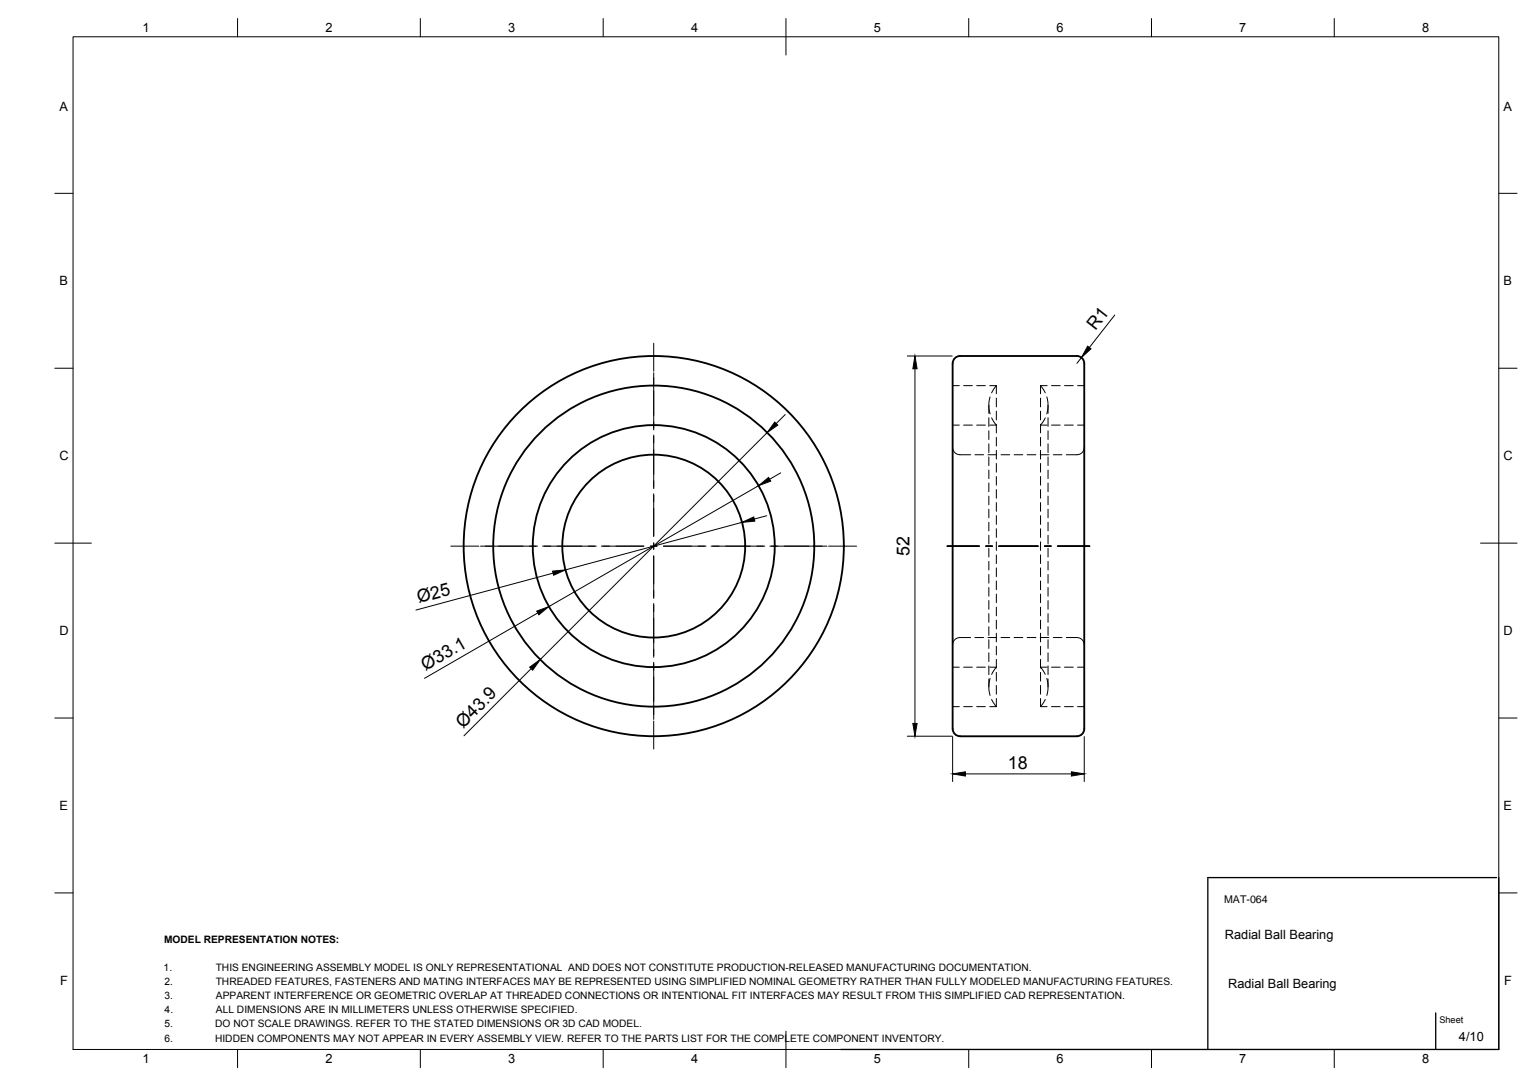
ISO-10303-21;
HEADER;
/* Generated by software containing ST-Developer
 * from STEP Tools, Inc. (www.steptools.com) 
 */

FILE_DESCRIPTION(
/* description */ (''),
/* implementation_level */ '2;1');

FILE_NAME(
/* name */ 
'Radial Ball Bearing.step',
/* time_stamp */ '2026-10-24T12:42:14-07:00',
/* author */ (''),
/* organization */ (''),
/* preprocessor_version */ 'ST-DEVELOPER v20.2',
/* originating_system */ 'Autodesk Translation Framework v15.15.0.0',
/* authorisation */ '');

FILE_SCHEMA (('AUTOMOTIVE_DESIGN { 1 0 10303 214 3 1 1 }'));
ENDSEC;

DATA;
#10=MECHANICAL_DESIGN_GEOMETRIC_PRESENTATION_REPRESENTATION('',(#69),#6789);
#57=SHAPE_REPRESENTATION_RELATIONSHIP('SRR','None',#6824,#63);
#63=ADVANCED_BREP_SHAPE_REPRESENTATION('',(#75),#6786);
#69=STYLED_ITEM('',(#6863),#75);
#75=MANIFOLD_SOLID_BREP('Radial Ball Bearing',#3964);
#86=TOROIDAL_SURFACE('',#4310,19.25,4.05);
#87=TOROIDAL_SURFACE('',#4324,13.5,1.);
#88=TOROIDAL_SURFACE('',#4329,13.5,1.);
#89=TOROIDAL_SURFACE('',#4333,19.25,4.05);
#90=TOROIDAL_SURFACE('',#4343,25.,0.999999999999999);
#91=TOROIDAL_SURFACE('',#4348,25.,0.999999999999999);
#161=CYLINDRICAL_SURFACE('',#4316,16.55);
#162=CYLINDRICAL_SURFACE('',#4318,16.55);
#163=CYLINDRICAL_SURFACE('',#4327,12.5);
#164=CYLINDRICAL_SURFACE('',#4337,21.95);
#165=CYLINDRICAL_SURFACE('',#4339,21.95);
#166=CYLINDRICAL_SURFACE('',#4346,26.);
#220=FACE_BOUND('',#813,.T.);
#221=FACE_BOUND('',#818,.T.);
#222=FACE_BOUND('',#823,.T.);
#223=FACE_BOUND('',#828,.T.);
#330=CIRCLE('',#4311,21.95);
#331=CIRCLE('',#4312,4.05);
#332=CIRCLE('',#4313,16.55);
#333=CIRCLE('',#4314,16.55);
#334=CIRCLE('',#4315,21.95);
#335=CIRCLE('',#4317,16.55);
#336=CIRCLE('',#4319,16.55);
#337=CIRCLE('',#4320,16.55);
#338=CIRCLE('',#4321,16.55);
#339=CIRCLE('',#4323,13.5);
#340=CIRCLE('',#4325,12.5);
#341=CIRCLE('',#4326,1.);
#342=CIRCLE('',#4328,12.5);
#343=CIRCLE('',#4330,13.5);
#344=CIRCLE('',#4331,1.);
#345=CIRCLE('',#4334,4.05);
#346=CIRCLE('',#4335,21.95);
#347=CIRCLE('',#4336,21.95);
#348=CIRCLE('',#4338,21.95);
#349=CIRCLE('',#4340,21.95);
#350=CIRCLE('',#4342,25.);
#351=CIRCLE('',#4344,0.999999999999999);
#352=CIRCLE('',#4345,26.);
#353=CIRCLE('',#4347,26.);
#354=CIRCLE('',#4349,0.999999999999999);
#355=CIRCLE('',#4350,25.);
#557=FACE_OUTER_BOUND('',#809,.T.);
#558=FACE_OUTER_BOUND('',#810,.T.);
#559=FACE_OUTER_BOUND('',#811,.T.);
#560=FACE_OUTER_BOUND('',#812,.T.);
#561=FACE_OUTER_BOUND('',#814,.T.);
#562=FACE_OUTER_BOUND('',#815,.T.);
#563=FACE_OUTER_BOUND('',#816,.T.);
#564=FACE_OUTER_BOUND('',#817,.T.);
#565=FACE_OUTER_BOUND('',#819,.T.);
#566=FACE_OUTER_BOUND('',#820,.T.);
#567=FACE_OUTER_BOUND('',#821,.T.);
#568=FACE_OUTER_BOUND('',#822,.T.);
#569=FACE_OUTER_BOUND('',#824,.T.);
#570=FACE_OUTER_BOUND('',#825,.T.);
#571=FACE_OUTER_BOUND('',#826,.T.);
#572=FACE_OUTER_BOUND('',#827,.T.);
#809=EDGE_LOOP('',(#3405,#3406,#3407,#3408,#3409,#3410));
#810=EDGE_LOOP('',(#3411,#3412,#3413,#3414,#3415));
#811=EDGE_LOOP('',(#3416,#3417,#3418,#3419,#3420));
#812=EDGE_LOOP('',(#3421));
#813=EDGE_LOOP('',(#3422));
#814=EDGE_LOOP('',(#3423,#3424,#3425,#3426));
#815=EDGE_LOOP('',(#3427,#3428,#3429,#3430));
#816=EDGE_LOOP('',(#3431,#3432,#3433,#3434));
#817=EDGE_LOOP('',(#3435));
#818=EDGE_LOOP('',(#3436));
#819=EDGE_LOOP('',(#3437,#3438,#3439,#3440,#3441,#3442));
#820=EDGE_LOOP('',(#3443,#3444,#3445,#3446,#3447));
#821=EDGE_LOOP('',(#3448,#3449,#3450,#3451,#3452));
#822=EDGE_LOOP('',(#3453));
#823=EDGE_LOOP('',(#3454));
#824=EDGE_LOOP('',(#3455,#3456,#3457,#3458));
#825=EDGE_LOOP('',(#3459,#3460,#3461,#3462));
#826=EDGE_LOOP('',(#3463,#3464,#3465,#3466));
#827=EDGE_LOOP('',(#3467));
#828=EDGE_LOOP('',(#3468));
#1217=LINE('',#6507,#1595);
#1218=LINE('',#6514,#1596);
#1219=LINE('',#6526,#1597);
#1220=LINE('',#6540,#1598);
#1221=LINE('',#6545,#1599);
#1222=LINE('',#6555,#1600);
#1595=VECTOR('',#5332,16.55);
#1596=VECTOR('',#5339,16.55);
#1597=VECTOR('',#5356,12.5);
#1598=VECTOR('',#5375,21.95);
#1599=VECTOR('',#5382,21.95);
#1600=VECTOR('',#5395,26.);
#1921=VERTEX_POINT('',#6495);
#1922=VERTEX_POINT('',#6496);
#1923=VERTEX_POINT('',#6498);
#1924=VERTEX_POINT('',#6500);
#1925=VERTEX_POINT('',#6505);
#1926=VERTEX_POINT('',#6509);
#1927=VERTEX_POINT('',#6510);
#1928=VERTEX_POINT('',#6513);
#1929=VERTEX_POINT('',#6517);
#1930=VERTEX_POINT('',#6520);
#1931=VERTEX_POINT('',#6524);
#1932=VERTEX_POINT('',#6528);
#1933=VERTEX_POINT('',#6533);
#1934=VERTEX_POINT('',#6535);
#1935=VERTEX_POINT('',#6539);
#1936=VERTEX_POINT('',#6543);
#1937=VERTEX_POINT('',#6547);
#1938=VERTEX_POINT('',#6550);
#1939=VERTEX_POINT('',#6554);
#1940=VERTEX_POINT('',#6558);
#2423=EDGE_CURVE('',#1921,#1922,#330,.F.);
#2424=EDGE_CURVE('',#1922,#1923,#331,.T.);
#2425=EDGE_CURVE('',#1923,#1924,#332,.T.);
#2426=EDGE_CURVE('',#1924,#1923,#333,.T.);
#2427=EDGE_CURVE('',#1922,#1921,#334,.F.);
#2428=EDGE_CURVE('',#1925,#1925,#335,.T.);
#2429=EDGE_CURVE('',#1925,#1924,#1217,.T.);
#2430=EDGE_CURVE('',#1926,#1927,#336,.T.);
#2431=EDGE_CURVE('',#1927,#1926,#337,.T.);
#2432=EDGE_CURVE('',#1927,#1928,#1218,.T.);
#2433=EDGE_CURVE('',#1928,#1928,#338,.T.);
#2434=EDGE_CURVE('',#1929,#1929,#339,.T.);
#2435=EDGE_CURVE('',#1930,#1930,#340,.T.);
#2436=EDGE_CURVE('',#1930,#1929,#341,.T.);
#2437=EDGE_CURVE('',#1931,#1931,#342,.T.);
#2438=EDGE_CURVE('',#1931,#1930,#1219,.T.);
#2439=EDGE_CURVE('',#1932,#1932,#343,.T.);
#2440=EDGE_CURVE('',#1932,#1931,#344,.T.);
#2441=EDGE_CURVE('',#1926,#1933,#345,.T.);
#2442=EDGE_CURVE('',#1933,#1934,#346,.F.);
#2443=EDGE_CURVE('',#1934,#1933,#347,.F.);
#2444=EDGE_CURVE('',#1921,#1935,#1220,.T.);
#2445=EDGE_CURVE('',#1935,#1935,#348,.T.);
#2446=EDGE_CURVE('',#1936,#1936,#349,.T.);
#2447=EDGE_CURVE('',#1936,#1934,#1221,.T.);
#2448=EDGE_CURVE('',#1937,#1937,#350,.T.);
#2449=EDGE_CURVE('',#1937,#1938,#351,.T.);
#2450=EDGE_CURVE('',#1938,#1938,#352,.T.);
#2451=EDGE_CURVE('',#1938,#1939,#1222,.T.);
#2452=EDGE_CURVE('',#1939,#1939,#353,.T.);
#2453=EDGE_CURVE('',#1939,#1940,#354,.T.);
#2454=EDGE_CURVE('',#1940,#1940,#355,.T.);
#3405=ORIENTED_EDGE('',*,*,#2423,.T.);
#3406=ORIENTED_EDGE('',*,*,#2424,.T.);
#3407=ORIENTED_EDGE('',*,*,#2425,.T.);
#3408=ORIENTED_EDGE('',*,*,#2426,.T.);
#3409=ORIENTED_EDGE('',*,*,#2424,.F.);
#3410=ORIENTED_EDGE('',*,*,#2427,.T.);
#3411=ORIENTED_EDGE('',*,*,#2428,.F.);
#3412=ORIENTED_EDGE('',*,*,#2429,.T.);
#3413=ORIENTED_EDGE('',*,*,#2425,.F.);
#3414=ORIENTED_EDGE('',*,*,#2426,.F.);
#3415=ORIENTED_EDGE('',*,*,#2429,.F.);
#3416=ORIENTED_EDGE('',*,*,#2430,.F.);
#3417=ORIENTED_EDGE('',*,*,#2431,.F.);
#3418=ORIENTED_EDGE('',*,*,#2432,.T.);
#3419=ORIENTED_EDGE('',*,*,#2433,.T.);
#3420=ORIENTED_EDGE('',*,*,#2432,.F.);
#3421=ORIENTED_EDGE('',*,*,#2428,.T.);
#3422=ORIENTED_EDGE('',*,*,#2434,.F.);
#3423=ORIENTED_EDGE('',*,*,#2435,.F.);
#3424=ORIENTED_EDGE('',*,*,#2436,.T.);
#3425=ORIENTED_EDGE('',*,*,#2434,.T.);
#3426=ORIENTED_EDGE('',*,*,#2436,.F.);
#3427=ORIENTED_EDGE('',*,*,#2437,.F.);
#3428=ORIENTED_EDGE('',*,*,#2438,.T.);
#3429=ORIENTED_EDGE('',*,*,#2435,.T.);
#3430=ORIENTED_EDGE('',*,*,#2438,.F.);
#3431=ORIENTED_EDGE('',*,*,#2439,.F.);
#3432=ORIENTED_EDGE('',*,*,#2440,.T.);
#3433=ORIENTED_EDGE('',*,*,#2437,.T.);
#3434=ORIENTED_EDGE('',*,*,#2440,.F.);
#3435=ORIENTED_EDGE('',*,*,#2433,.F.);
#3436=ORIENTED_EDGE('',*,*,#2439,.T.);
#3437=ORIENTED_EDGE('',*,*,#2430,.T.);
#3438=ORIENTED_EDGE('',*,*,#2431,.T.);
#3439=ORIENTED_EDGE('',*,*,#2441,.T.);
#3440=ORIENTED_EDGE('',*,*,#2442,.T.);
#3441=ORIENTED_EDGE('',*,*,#2443,.T.);
#3442=ORIENTED_EDGE('',*,*,#2441,.F.);
#3443=ORIENTED_EDGE('',*,*,#2423,.F.);
#3444=ORIENTED_EDGE('',*,*,#2444,.T.);
#3445=ORIENTED_EDGE('',*,*,#2445,.T.);
#3446=ORIENTED_EDGE('',*,*,#2444,.F.);
#3447=ORIENTED_EDGE('',*,*,#2427,.F.);
#3448=ORIENTED_EDGE('',*,*,#2446,.F.);
#3449=ORIENTED_EDGE('',*,*,#2447,.T.);
#3450=ORIENTED_EDGE('',*,*,#2442,.F.);
#3451=ORIENTED_EDGE('',*,*,#2443,.F.);
#3452=ORIENTED_EDGE('',*,*,#2447,.F.);
#3453=ORIENTED_EDGE('',*,*,#2448,.T.);
#3454=ORIENTED_EDGE('',*,*,#2445,.F.);
#3455=ORIENTED_EDGE('',*,*,#2448,.F.);
#3456=ORIENTED_EDGE('',*,*,#2449,.T.);
#3457=ORIENTED_EDGE('',*,*,#2450,.T.);
#3458=ORIENTED_EDGE('',*,*,#2449,.F.);
#3459=ORIENTED_EDGE('',*,*,#2450,.F.);
#3460=ORIENTED_EDGE('',*,*,#2451,.T.);
#3461=ORIENTED_EDGE('',*,*,#2452,.T.);
#3462=ORIENTED_EDGE('',*,*,#2451,.F.);
#3463=ORIENTED_EDGE('',*,*,#2452,.F.);
#3464=ORIENTED_EDGE('',*,*,#2453,.T.);
#3465=ORIENTED_EDGE('',*,*,#2454,.T.);
#3466=ORIENTED_EDGE('',*,*,#2453,.F.);
#3467=ORIENTED_EDGE('',*,*,#2454,.F.);
#3468=ORIENTED_EDGE('',*,*,#2446,.T.);
#3726=PLANE('',#4322);
#3727=PLANE('',#4332);
#3728=PLANE('',#4341);
#3729=PLANE('',#4351);
#3907=ADVANCED_FACE('',(#557),#86,.T.);
#3908=ADVANCED_FACE('',(#558),#161,.T.);
#3909=ADVANCED_FACE('',(#559),#162,.T.);
#3910=ADVANCED_FACE('',(#560,#220),#3726,.T.);
#3911=ADVANCED_FACE('',(#561),#87,.T.);
#3912=ADVANCED_FACE('',(#562),#163,.F.);
#3913=ADVANCED_FACE('',(#563),#88,.T.);
#3914=ADVANCED_FACE('',(#564,#221),#3727,.T.);
#3915=ADVANCED_FACE('',(#565),#89,.T.);
#3916=ADVANCED_FACE('',(#566),#164,.F.);
#3917=ADVANCED_FACE('',(#567),#165,.F.);
#3918=ADVANCED_FACE('',(#568,#222),#3728,.T.);
#3919=ADVANCED_FACE('',(#569),#90,.T.);
#3920=ADVANCED_FACE('',(#570),#166,.T.);
#3921=ADVANCED_FACE('',(#571),#91,.T.);
#3922=ADVANCED_FACE('',(#572,#223),#3729,.T.);
#3964=CLOSED_SHELL('',(#3907,#3908,#3909,#3910,#3911,#3912,#3913,#3914,
#3915,#3916,#3917,#3918,#3919,#3920,#3921,#3922));
#4309=AXIS2_PLACEMENT_3D('',#6493,#5314,#5315);
#4310=AXIS2_PLACEMENT_3D('',#6494,#5316,#5317);
#4311=AXIS2_PLACEMENT_3D('',#6497,#5318,#5319);
#4312=AXIS2_PLACEMENT_3D('',#6499,#5320,#5321);
#4313=AXIS2_PLACEMENT_3D('',#6501,#5322,#5323);
#4314=AXIS2_PLACEMENT_3D('',#6502,#5324,#5325);
#4315=AXIS2_PLACEMENT_3D('',#6503,#5326,#5327);
#4316=AXIS2_PLACEMENT_3D('',#6504,#5328,#5329);
#4317=AXIS2_PLACEMENT_3D('',#6506,#5330,#5331);
#4318=AXIS2_PLACEMENT_3D('',#6508,#5333,#5334);
#4319=AXIS2_PLACEMENT_3D('',#6511,#5335,#5336);
#4320=AXIS2_PLACEMENT_3D('',#6512,#5337,#5338);
#4321=AXIS2_PLACEMENT_3D('',#6515,#5340,#5341);
#4322=AXIS2_PLACEMENT_3D('',#6516,#5342,#5343);
#4323=AXIS2_PLACEMENT_3D('',#6518,#5344,#5345);
#4324=AXIS2_PLACEMENT_3D('',#6519,#5346,#5347);
#4325=AXIS2_PLACEMENT_3D('',#6521,#5348,#5349);
#4326=AXIS2_PLACEMENT_3D('',#6522,#5350,#5351);
#4327=AXIS2_PLACEMENT_3D('',#6523,#5352,#5353);
#4328=AXIS2_PLACEMENT_3D('',#6525,#5354,#5355);
#4329=AXIS2_PLACEMENT_3D('',#6527,#5357,#5358);
#4330=AXIS2_PLACEMENT_3D('',#6529,#5359,#5360);
#4331=AXIS2_PLACEMENT_3D('',#6530,#5361,#5362);
#4332=AXIS2_PLACEMENT_3D('',#6531,#5363,#5364);
#4333=AXIS2_PLACEMENT_3D('',#6532,#5365,#5366);
#4334=AXIS2_PLACEMENT_3D('',#6534,#5367,#5368);
#4335=AXIS2_PLACEMENT_3D('',#6536,#5369,#5370);
#4336=AXIS2_PLACEMENT_3D('',#6537,#5371,#5372);
#4337=AXIS2_PLACEMENT_3D('',#6538,#5373,#5374);
#4338=AXIS2_PLACEMENT_3D('',#6541,#5376,#5377);
#4339=AXIS2_PLACEMENT_3D('',#6542,#5378,#5379);
#4340=AXIS2_PLACEMENT_3D('',#6544,#5380,#5381);
#4341=AXIS2_PLACEMENT_3D('',#6546,#5383,#5384);
#4342=AXIS2_PLACEMENT_3D('',#6548,#5385,#5386);
#4343=AXIS2_PLACEMENT_3D('',#6549,#5387,#5388);
#4344=AXIS2_PLACEMENT_3D('',#6551,#5389,#5390);
#4345=AXIS2_PLACEMENT_3D('',#6552,#5391,#5392);
#4346=AXIS2_PLACEMENT_3D('',#6553,#5393,#5394);
#4347=AXIS2_PLACEMENT_3D('',#6556,#5396,#5397);
#4348=AXIS2_PLACEMENT_3D('',#6557,#5398,#5399);
#4349=AXIS2_PLACEMENT_3D('',#6559,#5400,#5401);
#4350=AXIS2_PLACEMENT_3D('',#6560,#5402,#5403);
#4351=AXIS2_PLACEMENT_3D('',#6561,#5404,#5405);
#5314=DIRECTION('axis',(0.,0.,1.));
#5315=DIRECTION('refdir',(1.,0.,0.));
#5316=DIRECTION('center_axis',(-1.,0.,0.));
#5317=DIRECTION('ref_axis',(0.,0.,1.));
#5318=DIRECTION('center_axis',(-1.,0.,0.));
#5319=DIRECTION('ref_axis',(0.,0.,1.));
#5320=DIRECTION('center_axis',(0.,-1.,1.22464679914735E-16));
#5321=DIRECTION('ref_axis',(0.,-1.22464679914735E-16,-1.));
#5322=DIRECTION('center_axis',(-1.,0.,0.));
#5323=DIRECTION('ref_axis',(0.,0.,1.));
#5324=DIRECTION('center_axis',(-1.,0.,0.));
#5325=DIRECTION('ref_axis',(0.,0.,1.));
#5326=DIRECTION('center_axis',(-1.,0.,0.));
#5327=DIRECTION('ref_axis',(0.,0.,1.));
#5328=DIRECTION('center_axis',(1.,0.,0.));
#5329=DIRECTION('ref_axis',(0.,0.,-1.));
#5330=DIRECTION('center_axis',(1.,0.,0.));
#5331=DIRECTION('ref_axis',(0.,0.,-1.));
#5332=DIRECTION('',(-1.,0.,0.));
#5333=DIRECTION('center_axis',(1.,0.,0.));
#5334=DIRECTION('ref_axis',(0.,0.,-1.));
#5335=DIRECTION('center_axis',(1.,0.,0.));
#5336=DIRECTION('ref_axis',(0.,0.,-1.));
#5337=DIRECTION('center_axis',(1.,0.,0.));
#5338=DIRECTION('ref_axis',(0.,0.,-1.));
#5339=DIRECTION('',(-1.,0.,0.));
#5340=DIRECTION('center_axis',(1.,0.,0.));
#5341=DIRECTION('ref_axis',(0.,0.,-1.));
#5342=DIRECTION('center_axis',(1.,0.,0.));
#5343=DIRECTION('ref_axis',(0.,0.,-1.));
#5344=DIRECTION('center_axis',(1.,0.,0.));
#5345=DIRECTION('ref_axis',(0.,0.,-1.));
#5346=DIRECTION('center_axis',(1.,0.,0.));
#5347=DIRECTION('ref_axis',(0.,0.,-1.));
#5348=DIRECTION('center_axis',(1.,0.,0.));
#5349=DIRECTION('ref_axis',(0.,0.,-1.));
#5350=DIRECTION('center_axis',(0.,-1.,-1.22464679914735E-16));
#5351=DIRECTION('ref_axis',(0.,-1.22464679914735E-16,1.));
#5352=DIRECTION('center_axis',(1.,0.,0.));
#5353=DIRECTION('ref_axis',(0.,0.,-1.));
#5354=DIRECTION('center_axis',(1.,0.,0.));
#5355=DIRECTION('ref_axis',(0.,0.,-1.));
#5356=DIRECTION('',(1.,0.,0.));
#5357=DIRECTION('center_axis',(1.,0.,0.));
#5358=DIRECTION('ref_axis',(0.,0.,-1.));
#5359=DIRECTION('center_axis',(1.,0.,0.));
#5360=DIRECTION('ref_axis',(0.,0.,-1.));
#5361=DIRECTION('center_axis',(0.,-1.,-1.22464679914735E-16));
#5362=DIRECTION('ref_axis',(0.,-1.22464679914735E-16,1.));
#5363=DIRECTION('center_axis',(-1.,0.,0.));
#5364=DIRECTION('ref_axis',(0.,0.,1.));
#5365=DIRECTION('center_axis',(-1.,0.,0.));
#5366=DIRECTION('ref_axis',(0.,0.,1.));
#5367=DIRECTION('center_axis',(0.,-1.,1.22464679914735E-16));
#5368=DIRECTION('ref_axis',(0.,-1.22464679914735E-16,-1.));
#5369=DIRECTION('center_axis',(1.,0.,0.));
#5370=DIRECTION('ref_axis',(0.,0.,-1.));
#5371=DIRECTION('center_axis',(1.,0.,0.));
#5372=DIRECTION('ref_axis',(0.,0.,-1.));
#5373=DIRECTION('center_axis',(1.,0.,0.));
#5374=DIRECTION('ref_axis',(0.,0.,-1.));
#5375=DIRECTION('',(1.,0.,0.));
#5376=DIRECTION('center_axis',(1.,0.,0.));
#5377=DIRECTION('ref_axis',(0.,0.,-1.));
#5378=DIRECTION('center_axis',(1.,0.,0.));
#5379=DIRECTION('ref_axis',(0.,0.,-1.));
#5380=DIRECTION('center_axis',(1.,0.,0.));
#5381=DIRECTION('ref_axis',(0.,0.,-1.));
#5382=DIRECTION('',(1.,0.,0.));
#5383=DIRECTION('center_axis',(1.,0.,0.));
#5384=DIRECTION('ref_axis',(0.,0.,-1.));
#5385=DIRECTION('center_axis',(1.,0.,0.));
#5386=DIRECTION('ref_axis',(0.,0.,-1.));
#5387=DIRECTION('center_axis',(1.,0.,0.));
#5388=DIRECTION('ref_axis',(0.,0.,-1.));
#5389=DIRECTION('center_axis',(0.,-1.,-1.22464679914735E-16));
#5390=DIRECTION('ref_axis',(0.,-1.22464679914735E-16,1.));
#5391=DIRECTION('center_axis',(1.,0.,0.));
#5392=DIRECTION('ref_axis',(0.,0.,-1.));
#5393=DIRECTION('center_axis',(1.,0.,0.));
#5394=DIRECTION('ref_axis',(0.,0.,-1.));
#5395=DIRECTION('',(-1.,0.,0.));
#5396=DIRECTION('center_axis',(1.,0.,0.));
#5397=DIRECTION('ref_axis',(0.,0.,-1.));
#5398=DIRECTION('center_axis',(1.,0.,0.));
#5399=DIRECTION('ref_axis',(0.,0.,-1.));
#5400=DIRECTION('center_axis',(0.,-1.,-1.22464679914735E-16));
#5401=DIRECTION('ref_axis',(0.,-1.22464679914735E-16,1.));
#5402=DIRECTION('center_axis',(1.,0.,0.));
#5403=DIRECTION('ref_axis',(0.,0.,-1.));
#5404=DIRECTION('center_axis',(-1.,0.,0.));
#5405=DIRECTION('ref_axis',(0.,0.,1.));
#6493=CARTESIAN_POINT('',(0.,0.,0.));
#6494=CARTESIAN_POINT('Origin',(0.,0.,0.));
#6495=CARTESIAN_POINT('',(3.01869176962471,0.,21.95));
#6496=CARTESIAN_POINT('',(3.01869176962471,-2.68809972412844E-15,-21.95));
#6497=CARTESIAN_POINT('Origin',(3.01869176962471,0.,0.));
#6498=CARTESIAN_POINT('',(3.01869176962472,-2.02679045258887E-15,-16.55));
#6499=CARTESIAN_POINT('Origin',(0.,-2.35744508835865E-15,-19.25));
#6500=CARTESIAN_POINT('',(3.01869176962472,0.,16.55));
#6501=CARTESIAN_POINT('Origin',(3.01869176962472,0.,0.));
#6502=CARTESIAN_POINT('Origin',(3.01869176962472,0.,0.));
#6503=CARTESIAN_POINT('Origin',(3.01869176962471,0.,0.));
#6504=CARTESIAN_POINT('Origin',(-20.6375,0.,0.));
#6505=CARTESIAN_POINT('',(9.,-2.02679045258887E-15,16.55));
#6506=CARTESIAN_POINT('Origin',(9.,0.,0.));
#6507=CARTESIAN_POINT('',(-20.6375,-2.02679045258887E-15,16.55));
#6508=CARTESIAN_POINT('Origin',(-20.6375,0.,0.));
#6509=CARTESIAN_POINT('',(-3.01869176962472,0.,-16.55));
#6510=CARTESIAN_POINT('',(-3.01869176962472,-2.02679045258887E-15,16.55));
#6511=CARTESIAN_POINT('Origin',(-3.01869176962472,0.,0.));
#6512=CARTESIAN_POINT('Origin',(-3.01869176962472,0.,0.));
#6513=CARTESIAN_POINT('',(-9.,-2.02679045258887E-15,16.55));
#6514=CARTESIAN_POINT('',(-20.6375,-2.02679045258887E-15,16.55));
#6515=CARTESIAN_POINT('Origin',(-9.,0.,0.));
#6516=CARTESIAN_POINT('Origin',(9.,13.5,0.));
#6517=CARTESIAN_POINT('',(9.,-1.65327317884893E-15,13.5));
#6518=CARTESIAN_POINT('Origin',(9.,0.,0.));
#6519=CARTESIAN_POINT('Origin',(8.,0.,0.));
#6520=CARTESIAN_POINT('',(8.,-1.53080849893419E-15,12.5));
#6521=CARTESIAN_POINT('Origin',(8.,0.,0.));
#6522=CARTESIAN_POINT('Origin',(8.,-1.65327317884893E-15,13.5));
#6523=CARTESIAN_POINT('Origin',(-20.6375,0.,0.));
#6524=CARTESIAN_POINT('',(-8.,-1.53080849893419E-15,12.5));
#6525=CARTESIAN_POINT('Origin',(-8.,0.,0.));
#6526=CARTESIAN_POINT('',(-20.6375,-1.53080849893419E-15,12.5));
#6527=CARTESIAN_POINT('Origin',(-8.,0.,0.));
#6528=CARTESIAN_POINT('',(-9.,-1.65327317884893E-15,13.5));
#6529=CARTESIAN_POINT('Origin',(-9.,0.,0.));
#6530=CARTESIAN_POINT('Origin',(-8.,-1.65327317884893E-15,13.5));
#6531=CARTESIAN_POINT('Origin',(-9.,16.55,0.));
#6532=CARTESIAN_POINT('Origin',(0.,0.,0.));
#6533=CARTESIAN_POINT('',(-3.01869176962471,0.,-21.95));
#6534=CARTESIAN_POINT('Origin',(0.,-2.35744508835865E-15,-19.25));
#6535=CARTESIAN_POINT('',(-3.01869176962471,-2.68809972412844E-15,21.95));
#6536=CARTESIAN_POINT('Origin',(-3.01869176962471,0.,0.));
#6537=CARTESIAN_POINT('Origin',(-3.01869176962471,0.,0.));
#6538=CARTESIAN_POINT('Origin',(-20.6375,0.,0.));
#6539=CARTESIAN_POINT('',(9.,-2.68809972412844E-15,21.95));
#6540=CARTESIAN_POINT('',(-20.6375,-2.68809972412844E-15,21.95));
#6541=CARTESIAN_POINT('Origin',(9.,0.,0.));
#6542=CARTESIAN_POINT('Origin',(-20.6375,0.,0.));
#6543=CARTESIAN_POINT('',(-9.,-2.68809972412844E-15,21.95));
#6544=CARTESIAN_POINT('Origin',(-9.,0.,0.));
#6545=CARTESIAN_POINT('',(-20.6375,-2.68809972412844E-15,21.95));
#6546=CARTESIAN_POINT('Origin',(9.,25.,0.));
#6547=CARTESIAN_POINT('',(9.,-3.06161699786838E-15,25.));
#6548=CARTESIAN_POINT('Origin',(9.,0.,0.));
#6549=CARTESIAN_POINT('Origin',(8.,0.,0.));
#6550=CARTESIAN_POINT('',(8.,-3.18408167778312E-15,26.));
#6551=CARTESIAN_POINT('Origin',(8.,-3.06161699786838E-15,25.));
#6552=CARTESIAN_POINT('Origin',(8.,0.,0.));
#6553=CARTESIAN_POINT('Origin',(-20.6375,0.,0.));
#6554=CARTESIAN_POINT('',(-8.,-3.18408167778312E-15,26.));
#6555=CARTESIAN_POINT('',(-20.6375,-3.18408167778312E-15,26.));
#6556=CARTESIAN_POINT('Origin',(-8.,0.,0.));
#6557=CARTESIAN_POINT('Origin',(-8.,0.,0.));
#6558=CARTESIAN_POINT('',(-9.,-3.06161699786838E-15,25.));
#6559=CARTESIAN_POINT('Origin',(-8.,-3.06161699786838E-15,25.));
#6560=CARTESIAN_POINT('Origin',(-9.,0.,0.));
#6561=CARTESIAN_POINT('Origin',(-9.,21.95,0.));
#6777=UNCERTAINTY_MEASURE_WITH_UNIT(LENGTH_MEASURE(0.01),#6790,
'DISTANCE_ACCURACY_VALUE',
'Maximum model space distance between geometric entities at asserted c
onnectivities');
#6780=UNCERTAINTY_MEASURE_WITH_UNIT(LENGTH_MEASURE(0.01),#6790,
'DISTANCE_ACCURACY_VALUE',
'Maximum model space distance between geometric entities at asserted c
onnectivities');
#6786=(
GEOMETRIC_REPRESENTATION_CONTEXT(3)
GLOBAL_UNCERTAINTY_ASSIGNED_CONTEXT((#6777))
GLOBAL_UNIT_ASSIGNED_CONTEXT((#6790,#6792,#6793))
REPRESENTATION_CONTEXT('','3D')
);
#6789=(
GEOMETRIC_REPRESENTATION_CONTEXT(3)
GLOBAL_UNCERTAINTY_ASSIGNED_CONTEXT((#6780))
GLOBAL_UNIT_ASSIGNED_CONTEXT((#6790,#6792,#6793))
REPRESENTATION_CONTEXT('','3D')
);
#6790=(
LENGTH_UNIT()
NAMED_UNIT(*)
SI_UNIT(.MILLI.,.METRE.)
);
#6792=(
NAMED_UNIT(*)
PLANE_ANGLE_UNIT()
SI_UNIT($,.RADIAN.)
);
#6793=(
NAMED_UNIT(*)
SI_UNIT($,.STERADIAN.)
SOLID_ANGLE_UNIT()
);
#6799=SHAPE_DEFINITION_REPRESENTATION(#6810,#6824);
#6810=PRODUCT_DEFINITION_SHAPE('',$,#6833);
#6824=SHAPE_REPRESENTATION('',(#4309),#6786);
#6827=PRODUCT_DEFINITION_CONTEXT('part definition',#6853,'design');
#6833=PRODUCT_DEFINITION('Radial Ball Bearing','Radial Ball Bearing',#6841,
#6827);
#6841=PRODUCT_DEFINITION_FORMATION('',$,#6860);
#6853=APPLICATION_CONTEXT(
'Core Data for Automotive Mechanical Design Process');
#6854=PRODUCT_CONTEXT('part definition',#6853,'mechanical');
#6860=PRODUCT('Radial Ball Bearing','Radial Ball Bearing',$,(#6854));
#6863=PRESENTATION_STYLE_ASSIGNMENT((#6865));
#6865=SURFACE_STYLE_USAGE(.BOTH.,#6867);
#6867=SURFACE_SIDE_STYLE('',(#6869));
#6869=SURFACE_STYLE_FILL_AREA(#6871);
#6871=FILL_AREA_STYLE('Steel - Satin',(#6873));
#6873=FILL_AREA_STYLE_COLOUR('Steel - Satin',#6875);
#6875=COLOUR_RGB('Steel - Satin',0.627450980392157,0.627450980392157,0.627450980392157);
ENDSEC;
END-ISO-10303-21;
